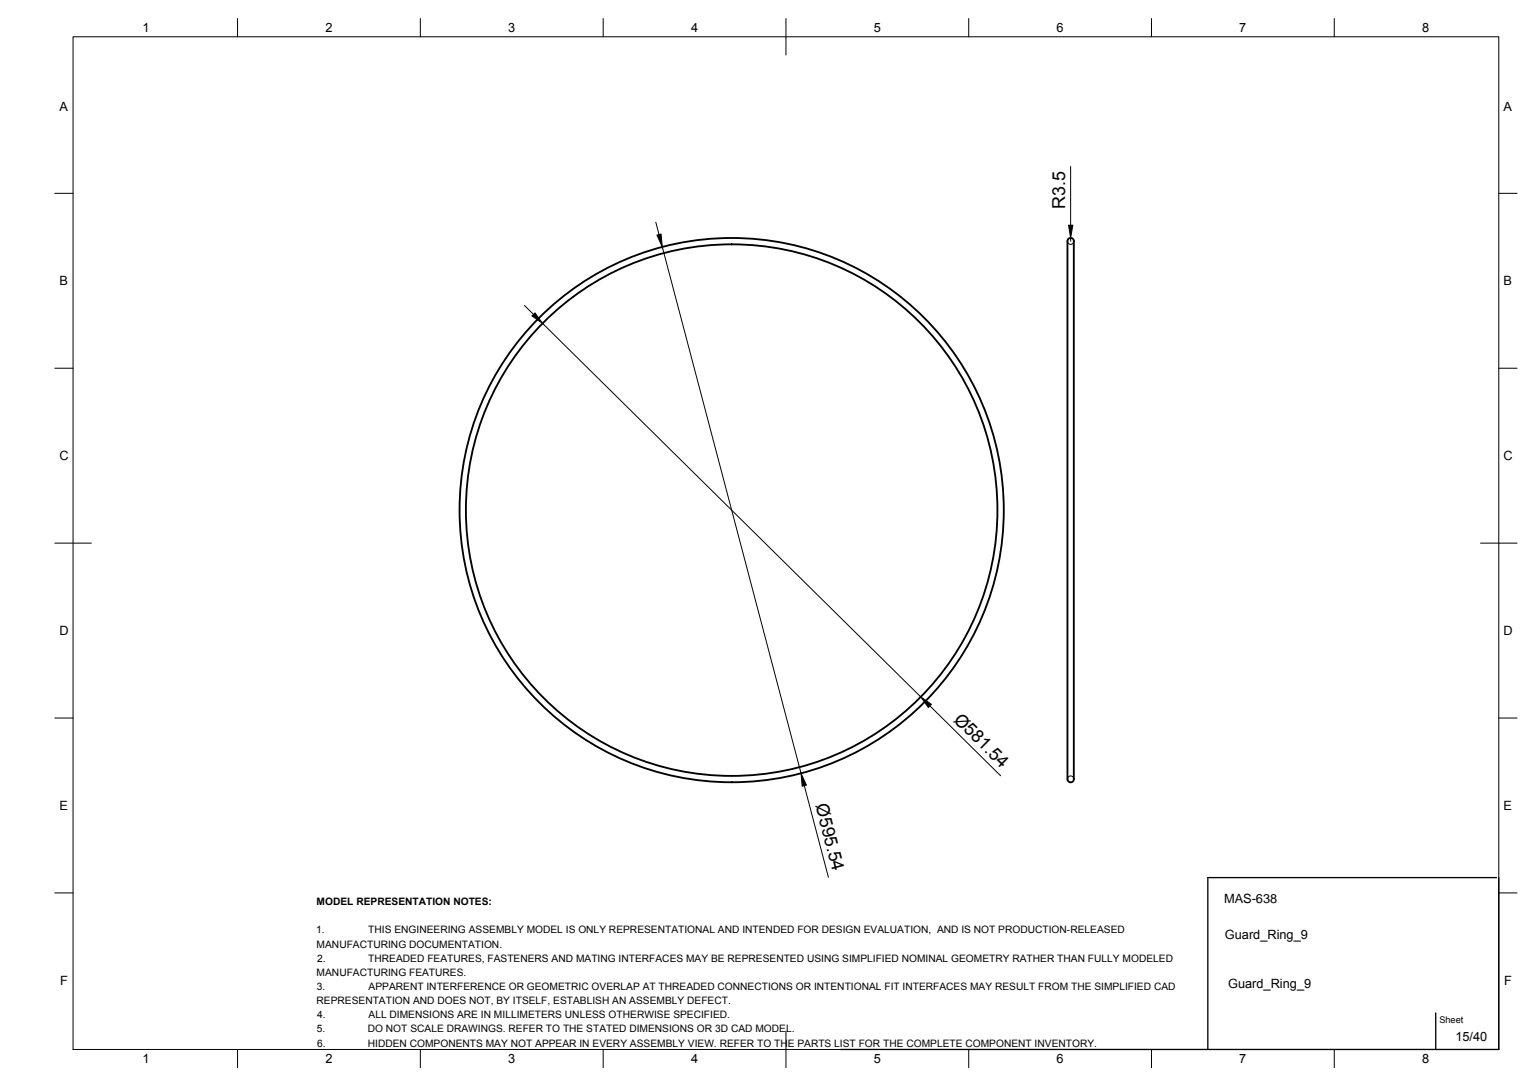
ISO-10303-21;
HEADER;
FILE_DESCRIPTION((''),'2;1');
FILE_NAME('Guard_Ring_9.step','2026-10-09T12:00:21-07:00',(''),(''),'','','');
FILE_SCHEMA (('AUTOMOTIVE_DESIGN { 1 0 10303 214 3 1 1 }'));
ENDSEC;
DATA;
#10=MECHANICAL_DESIGN_GEOMETRIC_PRESENTATION_REPRESENTATION('',(#407,#408),#10334);
#342=SHAPE_REPRESENTATION_RELATIONSHIP('SRR','None',#10458,#374) ;
#374=ADVANCED_BREP_SHAPE_REPRESENTATION('',(#446),#10310) ;
#407=STYLED_ITEM('',(#10631),#3375) ;
#408=STYLED_ITEM('',(#10632),#446) ;
#446=MANIFOLD_SOLID_BREP('Body1',#3568) ;
#867=FACE_OUTER_BOUND('',#1067,.T.) ;
#1067=EDGE_LOOP('',(#2381,#2382,#2383,#2384)) ;
#1292=CIRCLE('',#4007,0.349999999999999) ;
#1293=CIRCLE('',#4008,29.0768144613668) ;
#1521=VERTEX_POINT('',#5693) ;
#1847=EDGE_CURVE('',#1521,#1521,#1292,.T.) ;
#1848=EDGE_CURVE('',#1521,#1521,#1293,.T.) ;
#2381=ORIENTED_EDGE('',*,*,#1847,.F.) ;
#2382=ORIENTED_EDGE('',*,*,#1848,.T.) ;
#2383=ORIENTED_EDGE('',*,*,#1847,.T.) ;
#2384=ORIENTED_EDGE('',*,*,#1848,.F.) ;
#3313=TOROIDAL_SURFACE('',#4006,29.4268144613668,0.349999999999999) ;
#3375=ADVANCED_FACE('',(#867),#3313,.T.) ;
#3568=CLOSED_SHELL('',(#3375)) ;
#4005=AXIS2_PLACEMENT_3D('',#5691,#4571,#4572) ;
#4006=AXIS2_PLACEMENT_3D('',#5692,#4573,#4574) ;
#4007=AXIS2_PLACEMENT_3D('',#5694,#4575,#4576) ;
#4008=AXIS2_PLACEMENT_3D('',#5695,#4577,#4578) ;
#4571=DIRECTION('axis',(0.,0.,1.)) ;
#4572=DIRECTION('refdir',(1.,0.,0.)) ;
#4573=DIRECTION('center_axis',(-6.42891162084177E-17,-1.,-1.01883556321148E-16)) ;
#4574=DIRECTION('ref_axis',(1.,0.,0.)) ;
#4575=DIRECTION('center_axis',(0.,1.01883556321148E-16,-1.)) ;
#4576=DIRECTION('ref_axis',(-1.,0.,0.)) ;
#4577=DIRECTION('center_axis',(6.42891162084177E-17,1.,1.01883556321148E-16)) ;
#4578=DIRECTION('ref_axis',(1.,-6.42891162084177E-17,-6.55000379205715E-33)) ;
#5691=CARTESIAN_POINT('',(0.,0.,0.)) ;
#5692=CARTESIAN_POINT('Origin',(23.47768801576,67.3831179463143,68.2224337400009)) ;
#5693=CARTESIAN_POINT('',(-5.5991264456068,67.3831179463143,68.2224337400009)) ;
#5694=CARTESIAN_POINT('Origin',(-5.9491264456068,67.3831179463143,68.2224337400009)) ;
#5695=CARTESIAN_POINT('Origin',(23.47768801576,67.3831179463143,68.2224337400009)) ;
#10273=UNCERTAINTY_MEASURE_WITH_UNIT(LENGTH_MEASURE(0.001),#10335,
'DISTANCE_ACCURACY_VALUE',
'Maximum model space distance between geometric entities at asserted c
onnectivities') ;
#10297=UNCERTAINTY_MEASURE_WITH_UNIT(LENGTH_MEASURE(0.001),#10335,
'DISTANCE_ACCURACY_VALUE',
'Maximum model space distance between geometric entities at asserted c
onnectivities') ;
#10310=(
GEOMETRIC_REPRESENTATION_CONTEXT(3)
GLOBAL_UNCERTAINTY_ASSIGNED_CONTEXT((#10273))
GLOBAL_UNIT_ASSIGNED_CONTEXT((#10335,#10337,#10338))
REPRESENTATION_CONTEXT('','3D')
) ;
#10334=(
GEOMETRIC_REPRESENTATION_CONTEXT(3)
GLOBAL_UNCERTAINTY_ASSIGNED_CONTEXT((#10297))
GLOBAL_UNIT_ASSIGNED_CONTEXT((#10335,#10337,#10338))
REPRESENTATION_CONTEXT('','3D')
) ;
#10335=(
LENGTH_UNIT()
NAMED_UNIT(*)
SI_UNIT(.CENTI.,.METRE.)
) ;
#10337=(
NAMED_UNIT(*)
PLANE_ANGLE_UNIT()
SI_UNIT($,.RADIAN.)
) ;
#10338=(
NAMED_UNIT(*)
SI_UNIT($,.STERADIAN.)
SOLID_ANGLE_UNIT()
) ;
#10351=SHAPE_DEFINITION_REPRESENTATION(#10387,#10458) ;
#10387=PRODUCT_DEFINITION_SHAPE('',$,#10495) ;
#10458=SHAPE_REPRESENTATION('',(#4005),#10310) ;
#10482=PRODUCT_DEFINITION_CONTEXT('part definition',#10592,'design') ;
#10495=PRODUCT_DEFINITION('Guard_Ring_9','Guard_Ring_9',#10531,#10482) ;
#10531=PRODUCT_DEFINITION_FORMATION('',$,#10606) ;
#10592=APPLICATION_CONTEXT(
'Core Data for Automotive Mechanical Design Process') ;
#10593=PRODUCT_CONTEXT('part definition',#10592,'mechanical') ;
#10606=PRODUCT('Guard_Ring_9','Guard_Ring_9',$,(#10593)) ;
#10631=PRESENTATION_STYLE_ASSIGNMENT((#10635)) ;
#10632=PRESENTATION_STYLE_ASSIGNMENT((#10636)) ;
#10635=SURFACE_STYLE_USAGE(.BOTH.,#10639) ;
#10636=SURFACE_STYLE_USAGE(.BOTH.,#10640) ;
#10639=SURFACE_SIDE_STYLE('',(#10643)) ;
#10640=SURFACE_SIDE_STYLE('',(#10644)) ;
#10643=SURFACE_STYLE_FILL_AREA(#10647) ;
#10644=SURFACE_STYLE_FILL_AREA(#10648) ;
#10647=FILL_AREA_STYLE('Opaque(25,25,25)',(#10651)) ;
#10648=FILL_AREA_STYLE('Opaque(202,209,238)',(#10652)) ;
#10651=FILL_AREA_STYLE_COLOUR('Opaque(25,25,25)',#10655) ;
#10652=FILL_AREA_STYLE_COLOUR('Opaque(202,209,238)',#10656) ;
#10655=COLOUR_RGB('Opaque(25,25,25)', 0.09019608, 0.27058824, 0.51372549) ;
#10656=COLOUR_RGB('Opaque(202,209,238)', 0.40784314, 0.44705882, 0.49803922) ;
ENDSEC;
END-ISO-10303-21;
